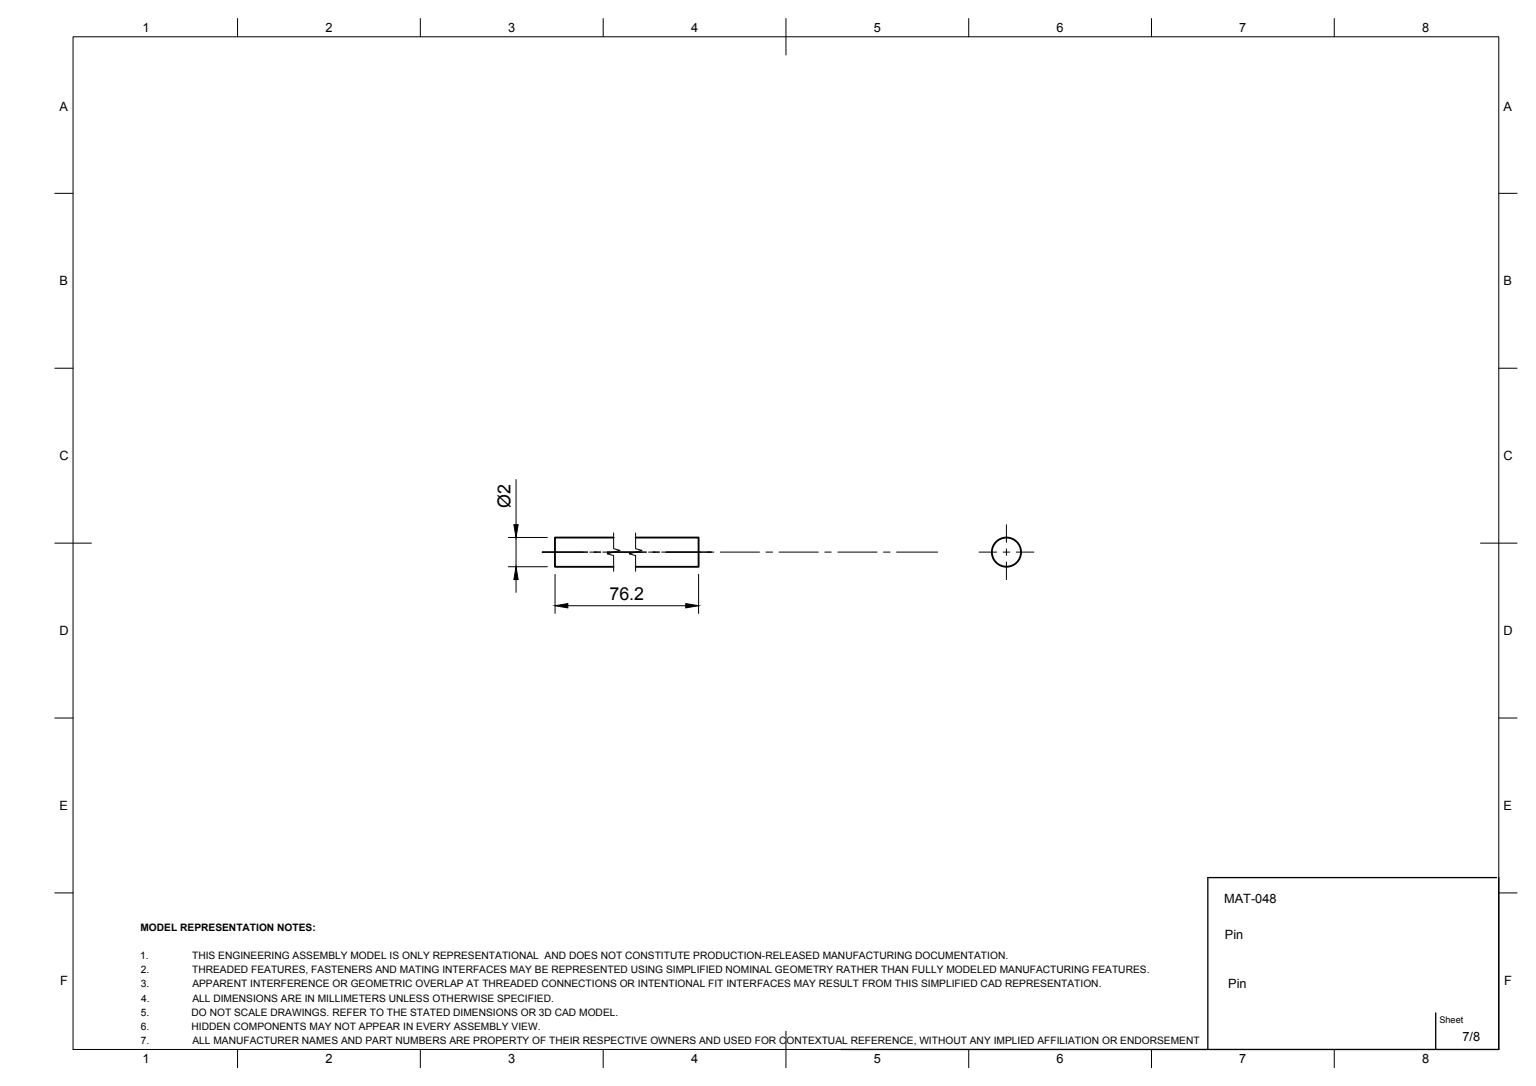
ISO-10303-21;
HEADER;
/* Generated by software containing ST-Developer
 * from STEP Tools, Inc. (www.steptools.com) 
 */

FILE_DESCRIPTION(
/* description */ ('STEP AP214'),
/* implementation_level */ '2;1');

FILE_NAME(
/* name */ 'Pin.step',
/* time_stamp */ '2026-11-14T22:24:45-08:00',
/* author */ (''),
/* organization */ (''),
/* preprocessor_version */ 'ST-DEVELOPER v20.2',
/* originating_system */ 'Autodesk Translation Framework v15.17.0.0',
/* authorisation */ '');

FILE_SCHEMA (('AUTOMOTIVE_DESIGN { 1 0 10303 214 3 1 1 }'));
ENDSEC;

DATA;
#10=MECHANICAL_DESIGN_GEOMETRIC_PRESENTATION_REPRESENTATION('',(#130),#5599);
#118=SHAPE_REPRESENTATION_RELATIONSHIP('SRR','None',#5646,#124);
#124=ADVANCED_BREP_SHAPE_REPRESENTATION('',(#136),#5598);
#130=STYLED_ITEM('',(#5680),#136);
#136=MANIFOLD_SOLID_BREP('Body1',#3312);
#192=CYLINDRICAL_SURFACE('',#3654,1.);
#279=CIRCLE('',#3655,1.);
#280=CIRCLE('',#3656,1.);
#454=FACE_OUTER_BOUND('',#644,.T.);
#455=FACE_OUTER_BOUND('',#645,.T.);
#456=FACE_OUTER_BOUND('',#646,.T.);
#644=EDGE_LOOP('',(#2997,#2998,#2999,#3000));
#645=EDGE_LOOP('',(#3001));
#646=EDGE_LOOP('',(#3002));
#1002=LINE('',#5558,#1358);
#1358=VECTOR('',#4588,1.);
#1645=VERTEX_POINT('',#5555);
#1646=VERTEX_POINT('',#5557);
#2096=EDGE_CURVE('',#1645,#1645,#279,.T.);
#2097=EDGE_CURVE('',#1645,#1646,#1002,.T.);
#2098=EDGE_CURVE('',#1646,#1646,#280,.T.);
#2997=ORIENTED_EDGE('',*,*,#2096,.T.);
#2998=ORIENTED_EDGE('',*,*,#2097,.T.);
#2999=ORIENTED_EDGE('',*,*,#2098,.F.);
#3000=ORIENTED_EDGE('',*,*,#2097,.F.);
#3001=ORIENTED_EDGE('',*,*,#2098,.T.);
#3002=ORIENTED_EDGE('',*,*,#2096,.F.);
#3129=PLANE('',#3657);
#3130=PLANE('',#3658);
#3304=ADVANCED_FACE('',(#454),#192,.T.);
#3305=ADVANCED_FACE('',(#455),#3129,.T.);
#3306=ADVANCED_FACE('',(#456),#3130,.F.);
#3312=CLOSED_SHELL('',(#3304,#3305,#3306));
#3653=AXIS2_PLACEMENT_3D('',#5553,#4582,#4583);
#3654=AXIS2_PLACEMENT_3D('',#5554,#4584,#4585);
#3655=AXIS2_PLACEMENT_3D('',#5556,#4586,#4587);
#3656=AXIS2_PLACEMENT_3D('',#5559,#4589,#4590);
#3657=AXIS2_PLACEMENT_3D('',#5560,#4591,#4592);
#3658=AXIS2_PLACEMENT_3D('',#5561,#4593,#4594);
#4582=DIRECTION('axis',(0.,0.,1.));
#4583=DIRECTION('refdir',(1.,0.,0.));
#4584=DIRECTION('center_axis',(4.99667015660473E-16,1.35737578475903E-15,
-1.));
#4585=DIRECTION('ref_axis',(-1.,5.55111512312586E-17,-4.99667015660472E-16));
#4586=DIRECTION('center_axis',(-4.99667015660473E-16,-1.35737578475903E-15,
1.));
#4587=DIRECTION('ref_axis',(1.,-5.55111512312592E-17,4.99667015660473E-16));
#4588=DIRECTION('',(-4.99667015660473E-16,-1.35737578475903E-15,1.));
#4589=DIRECTION('center_axis',(-4.99667015660473E-16,-1.35737578475903E-15,
1.));
#4590=DIRECTION('ref_axis',(1.,-5.55111512312586E-17,4.99667015660473E-16));
#4591=DIRECTION('center_axis',(4.99667015660476E-16,-1.35737578475903E-15,
1.));
#4592=DIRECTION('ref_axis',(1.,-5.55111512312578E-17,-4.99667015660476E-16));
#4593=DIRECTION('center_axis',(4.99667015660476E-16,-1.35737578475903E-15,
1.));
#4594=DIRECTION('ref_axis',(1.,-5.55111512312578E-17,-4.99667015660476E-16));
#5553=CARTESIAN_POINT('',(0.,0.,0.));
#5554=CARTESIAN_POINT('Origin',(-1.38777878078145E-14,-1.38777878078145E-14,
76.2000000000004));
#5555=CARTESIAN_POINT('',(1.00000000000002,8.93762711596783E-14,0.));
#5556=CARTESIAN_POINT('Origin',(0.,0.,0.));
#5557=CARTESIAN_POINT('',(0.999999999999986,-1.40557636389605E-14,76.2000000000004));
#5558=CARTESIAN_POINT('',(0.999999999999986,-1.40557636389605E-14,76.2000000000004));
#5559=CARTESIAN_POINT('Origin',(-1.38777878078145E-14,-1.38777878078145E-14,
76.2000000000004));
#5560=CARTESIAN_POINT('Origin',(-1.38777878078145E-14,-1.38777878078145E-14,
76.2000000000004));
#5561=CARTESIAN_POINT('Origin',(0.,0.,0.));
#5590=UNCERTAINTY_MEASURE_WITH_UNIT(LENGTH_MEASURE(0.01),#5600,
'DISTANCE_ACCURACY_VALUE',
'Maximum model space distance between geometric entities at asserted c
onnectivities');
#5591=UNCERTAINTY_MEASURE_WITH_UNIT(LENGTH_MEASURE(0.01),#5600,
'DISTANCE_ACCURACY_VALUE',
'Maximum model space distance between geometric entities at asserted c
onnectivities');
#5598=(
GEOMETRIC_REPRESENTATION_CONTEXT(3)
GLOBAL_UNCERTAINTY_ASSIGNED_CONTEXT((#5590))
GLOBAL_UNIT_ASSIGNED_CONTEXT((#5600,#5602,#5603))
REPRESENTATION_CONTEXT('','3D')
);
#5599=(
GEOMETRIC_REPRESENTATION_CONTEXT(3)
GLOBAL_UNCERTAINTY_ASSIGNED_CONTEXT((#5591))
GLOBAL_UNIT_ASSIGNED_CONTEXT((#5600,#5602,#5603))
REPRESENTATION_CONTEXT('','3D')
);
#5600=(
LENGTH_UNIT()
NAMED_UNIT(*)
SI_UNIT(.MILLI.,.METRE.)
);
#5602=(
NAMED_UNIT(*)
PLANE_ANGLE_UNIT()
SI_UNIT($,.RADIAN.)
);
#5603=(
NAMED_UNIT(*)
SI_UNIT($,.STERADIAN.)
SOLID_ANGLE_UNIT()
);
#5610=SHAPE_DEFINITION_REPRESENTATION(#5617,#5646);
#5617=PRODUCT_DEFINITION_SHAPE('',$,#5654);
#5646=SHAPE_REPRESENTATION('',(#3653),#5598);
#5647=PRODUCT_DEFINITION_CONTEXT('part definition',#5670,'design');
#5654=PRODUCT_DEFINITION('Pin','Pin',#5661,#5647);
#5661=PRODUCT_DEFINITION_FORMATION('',$,#5678);
#5670=APPLICATION_CONTEXT(
'Core Data for Automotive Mechanical Design Process');
#5671=PRODUCT_CONTEXT('part definition',#5670,'mechanical');
#5678=PRODUCT('Pin','Pin',$,(#5671));
#5680=PRESENTATION_STYLE_ASSIGNMENT((#5683));
#5683=SURFACE_STYLE_USAGE(.BOTH.,#5686);
#5686=SURFACE_SIDE_STYLE('',(#5689));
#5689=SURFACE_STYLE_FILL_AREA(#5692);
#5692=FILL_AREA_STYLE('Opaque(97,158,199)',(#5695));
#5695=FILL_AREA_STYLE_COLOUR('Opaque(97,158,199)',#5698);
#5698=COLOUR_RGB('Opaque(97,158,199)',0.380392156862745,0.619607843137255,
0.780392156862745);
ENDSEC;
END-ISO-10303-21;
